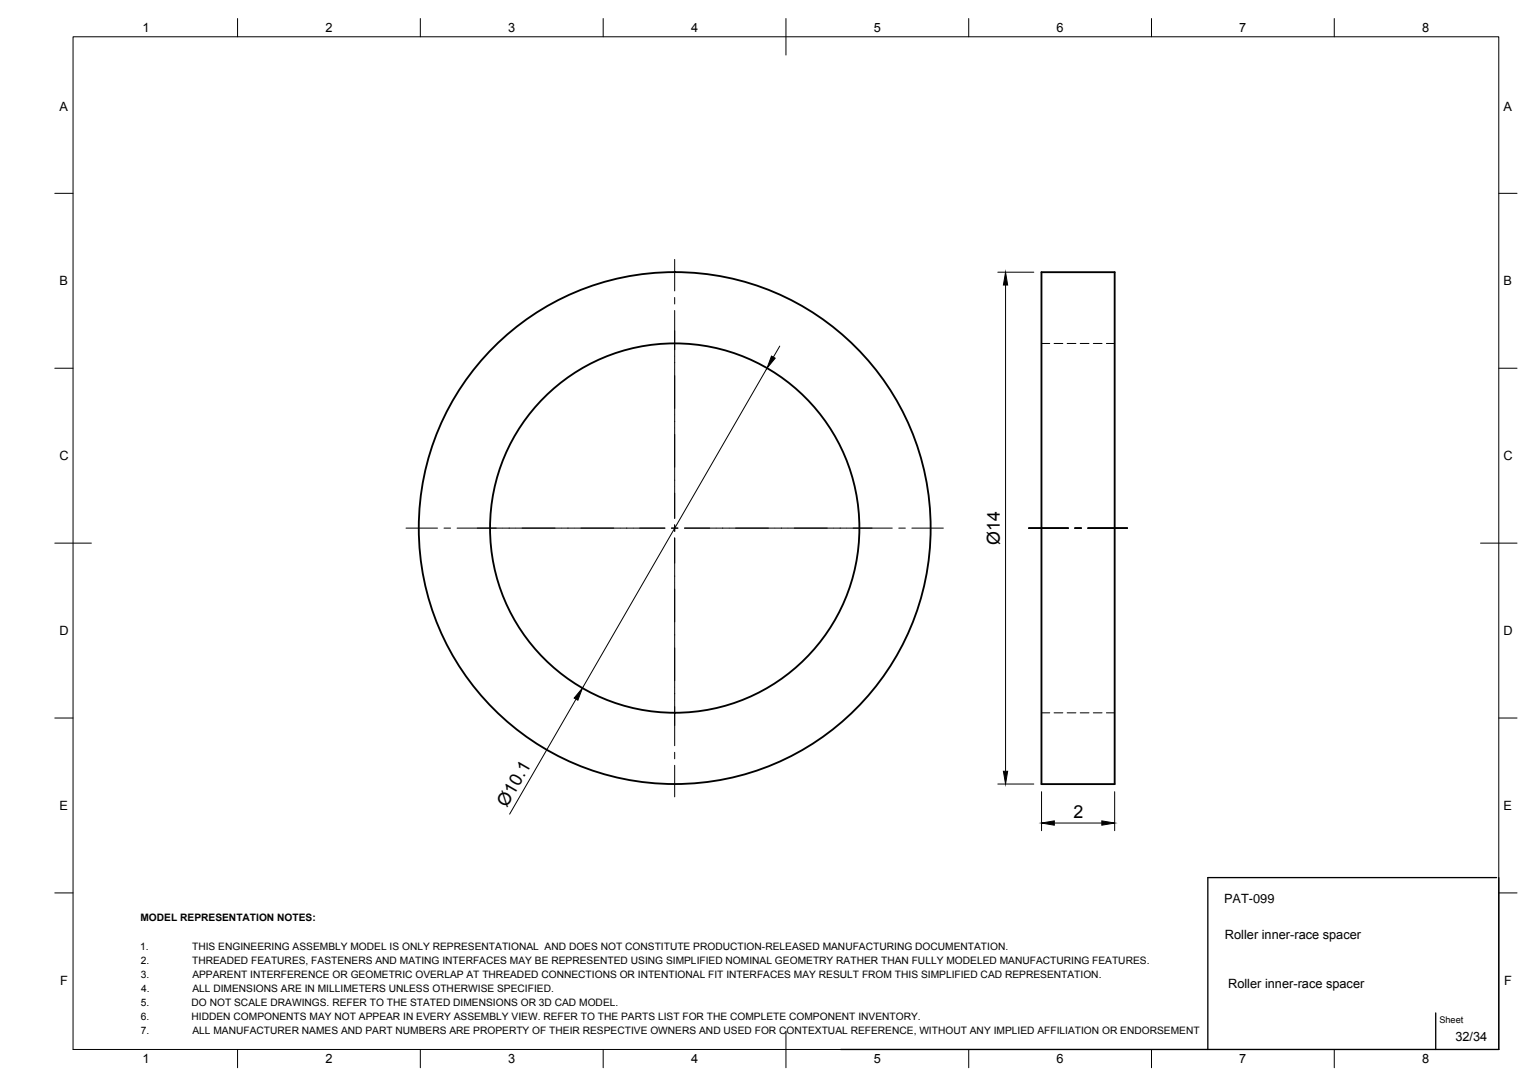
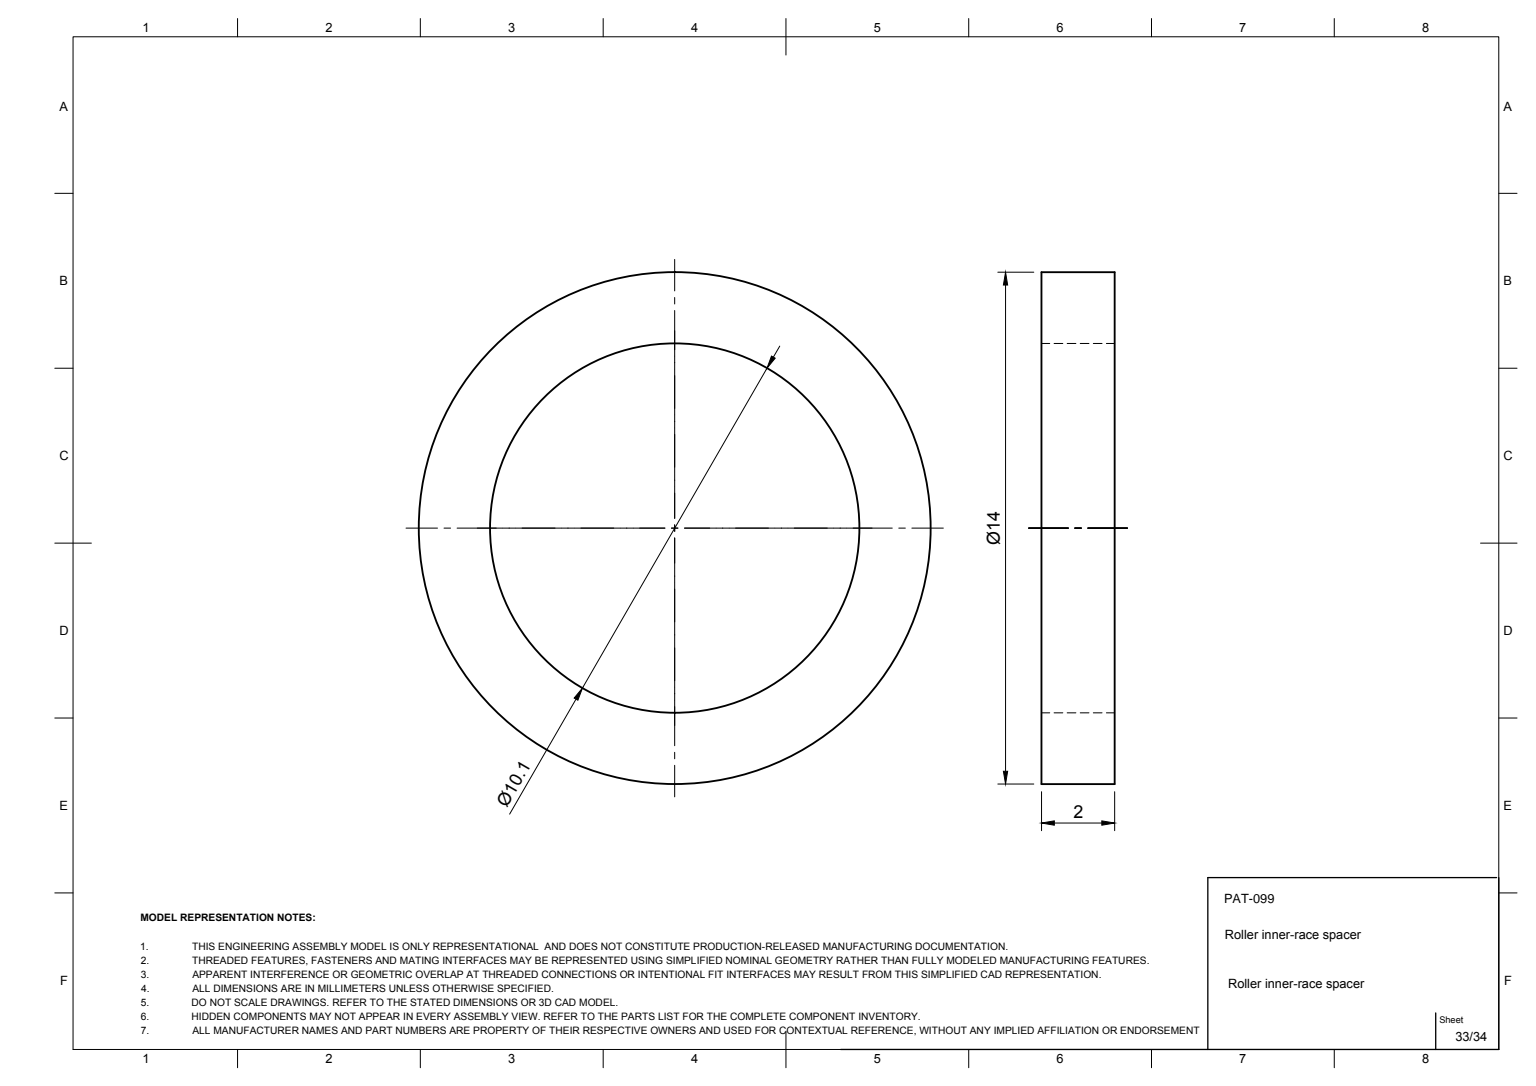
ISO-10303-21;
HEADER;
/* Generated by software containing ST-Developer
 * from STEP Tools, Inc. (www.steptools.com) 
 */

FILE_DESCRIPTION(
/* description */ ('PAT-099'),
/* implementation_level */ '2;1');

FILE_NAME(
/* name */ 'Roller inner-race spacer.step',
/* time_stamp */ '2026-10-29T17:25:42-07:00',
/* author */ (''),
/* organization */ (''),
/* preprocessor_version */ 'ST-DEVELOPER v20.2',
/* originating_system */ 'Autodesk Translation Framework v15.17.0.0',
/* authorisation */ '');

FILE_SCHEMA (('AUTOMOTIVE_DESIGN { 1 0 10303 214 3 1 1 }'));
ENDSEC;

DATA;
#10=MECHANICAL_DESIGN_GEOMETRIC_PRESENTATION_REPRESENTATION('',(#353),#11035);
#303=SHAPE_REPRESENTATION_RELATIONSHIP('SRR','None',#11174,#328);
#328=ADVANCED_BREP_SHAPE_REPRESENTATION('',(#385),#11024);
#353=STYLED_ITEM('',(#11379),#385);
#385=MANIFOLD_SOLID_BREP('Body1',#4722);
#507=FACE_BOUND('',#1251,.T.);
#508=FACE_BOUND('',#1253,.T.);
#625=PLANE('',#5451);
#626=PLANE('',#5452);
#861=FACE_OUTER_BOUND('',#1248,.T.);
#862=FACE_OUTER_BOUND('',#1249,.T.);
#863=FACE_OUTER_BOUND('',#1250,.T.);
#864=FACE_OUTER_BOUND('',#1252,.T.);
#1248=EDGE_LOOP('',(#4001,#4002,#4003,#4004));
#1249=EDGE_LOOP('',(#4005,#4006,#4007,#4008));
#1250=EDGE_LOOP('',(#4009));
#1251=EDGE_LOOP('',(#4010));
#1252=EDGE_LOOP('',(#4011));
#1253=EDGE_LOOP('',(#4012));
#1550=LINE('',#10239,#1802);
#1551=LINE('',#10245,#1803);
#1802=VECTOR('',#6737,0.505);
#1803=VECTOR('',#6744,0.7);
#2047=CIRCLE('',#5446,0.505);
#2048=CIRCLE('',#5447,0.505);
#2049=CIRCLE('',#5449,0.7);
#2050=CIRCLE('',#5450,0.7);
#2431=VERTEX_POINT('',#10236);
#2432=VERTEX_POINT('',#10238);
#2433=VERTEX_POINT('',#10242);
#2434=VERTEX_POINT('',#10244);
#2977=EDGE_CURVE('',#2431,#2431,#2047,.T.);
#2978=EDGE_CURVE('',#2431,#2432,#1550,.T.);
#2979=EDGE_CURVE('',#2432,#2432,#2048,.T.);
#2980=EDGE_CURVE('',#2433,#2433,#2049,.T.);
#2981=EDGE_CURVE('',#2433,#2434,#1551,.T.);
#2982=EDGE_CURVE('',#2434,#2434,#2050,.T.);
#4001=ORIENTED_EDGE('',*,*,#2977,.F.);
#4002=ORIENTED_EDGE('',*,*,#2978,.T.);
#4003=ORIENTED_EDGE('',*,*,#2979,.T.);
#4004=ORIENTED_EDGE('',*,*,#2978,.F.);
#4005=ORIENTED_EDGE('',*,*,#2980,.F.);
#4006=ORIENTED_EDGE('',*,*,#2981,.T.);
#4007=ORIENTED_EDGE('',*,*,#2982,.T.);
#4008=ORIENTED_EDGE('',*,*,#2981,.F.);
#4009=ORIENTED_EDGE('',*,*,#2980,.T.);
#4010=ORIENTED_EDGE('',*,*,#2977,.T.);
#4011=ORIENTED_EDGE('',*,*,#2982,.F.);
#4012=ORIENTED_EDGE('',*,*,#2979,.F.);
#4404=CYLINDRICAL_SURFACE('',#5445,0.505);
#4405=CYLINDRICAL_SURFACE('',#5448,0.7);
#4626=ADVANCED_FACE('',(#861),#4404,.F.);
#4627=ADVANCED_FACE('',(#862),#4405,.T.);
#4628=ADVANCED_FACE('',(#863,#507),#625,.T.);
#4629=ADVANCED_FACE('',(#864,#508),#626,.F.);
#4722=CLOSED_SHELL('',(#4626,#4627,#4628,#4629));
#5444=AXIS2_PLACEMENT_3D('',#10234,#6731,#6732);
#5445=AXIS2_PLACEMENT_3D('',#10235,#6733,#6734);
#5446=AXIS2_PLACEMENT_3D('',#10237,#6735,#6736);
#5447=AXIS2_PLACEMENT_3D('',#10240,#6738,#6739);
#5448=AXIS2_PLACEMENT_3D('',#10241,#6740,#6741);
#5449=AXIS2_PLACEMENT_3D('',#10243,#6742,#6743);
#5450=AXIS2_PLACEMENT_3D('',#10246,#6745,#6746);
#5451=AXIS2_PLACEMENT_3D('',#10247,#6747,#6748);
#5452=AXIS2_PLACEMENT_3D('',#10248,#6749,#6750);
#6731=DIRECTION('axis',(0.,0.,1.));
#6732=DIRECTION('refdir',(1.,0.,0.));
#6733=DIRECTION('center_axis',(0.,0.,1.));
#6734=DIRECTION('ref_axis',(1.,0.,0.));
#6735=DIRECTION('center_axis',(0.,0.,-1.));
#6736=DIRECTION('ref_axis',(1.,0.,0.));
#6737=DIRECTION('',(0.,0.,-1.));
#6738=DIRECTION('center_axis',(0.,0.,-1.));
#6739=DIRECTION('ref_axis',(1.,0.,0.));
#6740=DIRECTION('center_axis',(0.,0.,1.));
#6741=DIRECTION('ref_axis',(1.,0.,0.));
#6742=DIRECTION('center_axis',(0.,0.,1.));
#6743=DIRECTION('ref_axis',(1.,0.,0.));
#6744=DIRECTION('',(0.,0.,-1.));
#6745=DIRECTION('center_axis',(0.,0.,1.));
#6746=DIRECTION('ref_axis',(1.,0.,0.));
#6747=DIRECTION('center_axis',(0.,0.,1.));
#6748=DIRECTION('ref_axis',(1.,0.,0.));
#6749=DIRECTION('center_axis',(0.,0.,1.));
#6750=DIRECTION('ref_axis',(1.,0.,0.));
#10234=CARTESIAN_POINT('',(0.,0.,0.));
#10235=CARTESIAN_POINT('Origin',(4.,0.,4.6));
#10236=CARTESIAN_POINT('',(3.495,-6.18446633569413E-17,4.8));
#10237=CARTESIAN_POINT('Origin',(4.,0.,4.8));
#10238=CARTESIAN_POINT('',(3.495,-6.18446633569413E-17,4.6));
#10239=CARTESIAN_POINT('',(3.495,-6.18446633569413E-17,4.6));
#10240=CARTESIAN_POINT('Origin',(4.,0.,4.6));
#10241=CARTESIAN_POINT('Origin',(4.,0.,4.6));
#10242=CARTESIAN_POINT('',(3.3,-8.57252759403147E-17,4.8));
#10243=CARTESIAN_POINT('Origin',(4.,0.,4.8));
#10244=CARTESIAN_POINT('',(3.3,-8.57252759403147E-17,4.6));
#10245=CARTESIAN_POINT('',(3.3,-8.57252759403147E-17,4.6));
#10246=CARTESIAN_POINT('Origin',(4.,0.,4.6));
#10247=CARTESIAN_POINT('Origin',(4.,0.,4.8));
#10248=CARTESIAN_POINT('Origin',(4.,0.,4.6));
#10991=UNCERTAINTY_MEASURE_WITH_UNIT(LENGTH_MEASURE(0.001),#11036,
'DISTANCE_ACCURACY_VALUE',
'Maximum model space distance between geometric entities at asserted c
onnectivities');
#11002=UNCERTAINTY_MEASURE_WITH_UNIT(LENGTH_MEASURE(0.001),#11036,
'DISTANCE_ACCURACY_VALUE',
'Maximum model space distance between geometric entities at asserted c
onnectivities');
#11024=(
GEOMETRIC_REPRESENTATION_CONTEXT(3)
GLOBAL_UNCERTAINTY_ASSIGNED_CONTEXT((#10991))
GLOBAL_UNIT_ASSIGNED_CONTEXT((#11036,#11038,#11039))
REPRESENTATION_CONTEXT('','3D')
);
#11035=(
GEOMETRIC_REPRESENTATION_CONTEXT(3)
GLOBAL_UNCERTAINTY_ASSIGNED_CONTEXT((#11002))
GLOBAL_UNIT_ASSIGNED_CONTEXT((#11036,#11038,#11039))
REPRESENTATION_CONTEXT('','3D')
);
#11036=(
LENGTH_UNIT()
NAMED_UNIT(*)
SI_UNIT(.CENTI.,.METRE.)
);
#11038=(
NAMED_UNIT(*)
PLANE_ANGLE_UNIT()
SI_UNIT($,.RADIAN.)
);
#11039=(
NAMED_UNIT(*)
SI_UNIT($,.STERADIAN.)
SOLID_ANGLE_UNIT()
);
#11061=SHAPE_DEFINITION_REPRESENTATION(#11099,#11174);
#11099=PRODUCT_DEFINITION_SHAPE('',$,#11207);
#11174=SHAPE_REPRESENTATION('',(#5444),#11024);
#11185=PRODUCT_DEFINITION_CONTEXT('part definition',#11283,'design');
#11207=PRODUCT_DEFINITION('Roller inner-race spacer',
'Roller inner-race spacer',#11239,#11185);
#11239=PRODUCT_DEFINITION_FORMATION('',$,#11306);
#11283=APPLICATION_CONTEXT(
'Core Data for Automotive Mechanical Design Process');
#11284=PRODUCT_CONTEXT('part definition',#11283,'mechanical');
#11306=PRODUCT('Roller inner-race spacer','Roller inner-race spacer',
'Roller inner-race spacer',(#11284));
#11373=COLOUR_RGB('Sky Blue',0.24,0.69,0.87);
#11374=FILL_AREA_STYLE_COLOUR('',#11373);
#11375=FILL_AREA_STYLE('',(#11374));
#11376=SURFACE_STYLE_FILL_AREA(#11375);
#11377=SURFACE_SIDE_STYLE('',(#11376));
#11378=SURFACE_STYLE_USAGE(.BOTH.,#11377);
#11379=PRESENTATION_STYLE_ASSIGNMENT((#11378));
ENDSEC;
END-ISO-10303-21;
